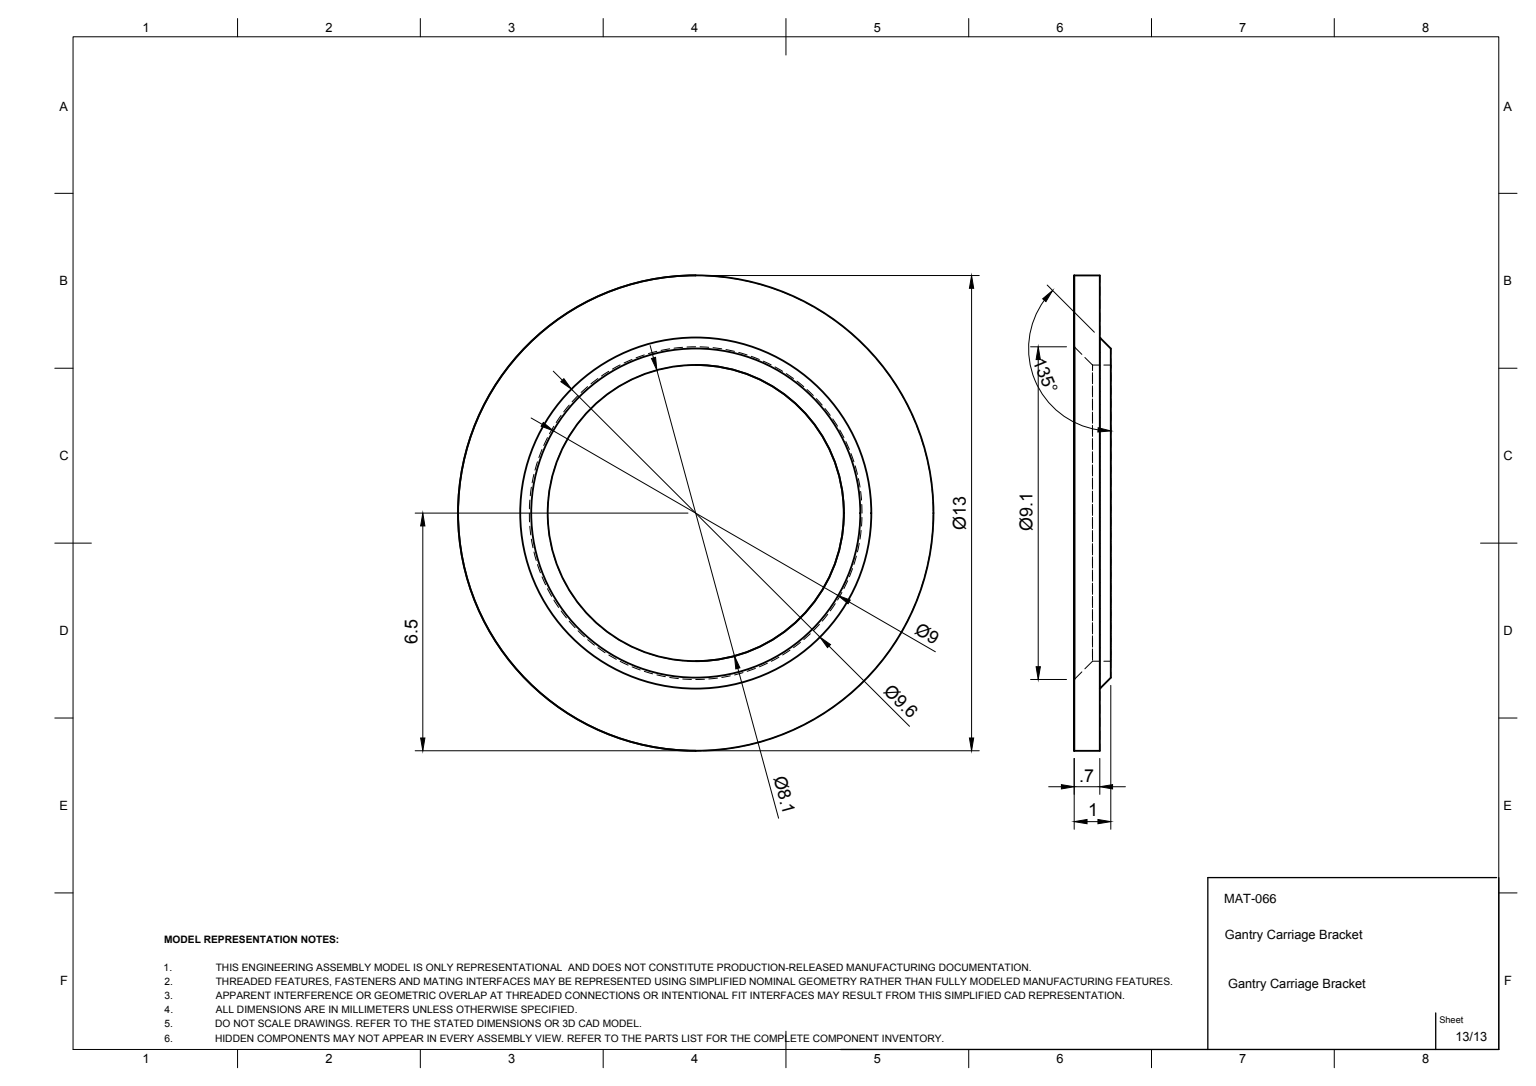
ISO-10303-21;
HEADER;
/* Generated by software containing ST-Developer
 * from STEP Tools, Inc. (www.steptools.com) 
 */

FILE_DESCRIPTION(
/* description */ ('CAx-IF Rec.Pracs.---Representation and Presentation of Product Manufa
cturing Information (PMI)---4.0---2014-10-13'),
/* implementation_level */ '2;1');

FILE_NAME(
/* name */ 'Gantry Carriage Bracket.step',
/* time_stamp */ '2026-10-24T15:58:00-07:00',
/* author */ (''),
/* organization */ (''),
/* preprocessor_version */ 'ST-DEVELOPER v20.2',
/* originating_system */ 'Autodesk Translation Framework v15.17.0.0',
/* authorisation */ '');

FILE_SCHEMA (('AP242_MANAGED_MODEL_BASED_3D_ENGINEERING_MIM_LF { 1 0 10303 442 2 1 4 }'));
ENDSEC;

DATA;
#10=MECHANICAL_DESIGN_GEOMETRIC_PRESENTATION_REPRESENTATION('',(#137),#8944);
#107=CONICAL_SURFACE('',#5788,0.0043,0.785398163397448);
#108=CONICAL_SURFACE('',#5794,0.0046499998960644,0.785398163397448);
#119=SHAPE_REPRESENTATION_RELATIONSHIP('SRR','None',#9002,#128);
#128=ADVANCED_BREP_SHAPE_REPRESENTATION('',(#146),#8943);
#137=STYLED_ITEM('',(#9052),#146);
#146=MANIFOLD_SOLID_BREP('Body1',#5158);
#236=CYLINDRICAL_SURFACE('',#5784,0.0065);
#237=CYLINDRICAL_SURFACE('',#5790,0.00405);
#305=FACE_BOUND('',#907,.T.);
#306=FACE_BOUND('',#910,.T.);
#307=FACE_BOUND('',#914,.T.);
#570=FACE_OUTER_BOUND('',#906,.T.);
#571=FACE_OUTER_BOUND('',#908,.T.);
#572=FACE_OUTER_BOUND('',#909,.T.);
#573=FACE_OUTER_BOUND('',#911,.T.);
#574=FACE_OUTER_BOUND('',#912,.T.);
#575=FACE_OUTER_BOUND('',#913,.T.);
#576=FACE_OUTER_BOUND('',#915,.T.);
#906=EDGE_LOOP('',(#4687));
#907=EDGE_LOOP('',(#4688));
#908=EDGE_LOOP('',(#4689,#4690,#4691,#4692));
#909=EDGE_LOOP('',(#4693));
#910=EDGE_LOOP('',(#4694));
#911=EDGE_LOOP('',(#4695,#4696,#4697,#4698));
#912=EDGE_LOOP('',(#4699,#4700,#4701,#4702));
#913=EDGE_LOOP('',(#4703));
#914=EDGE_LOOP('',(#4704));
#915=EDGE_LOOP('',(#4705,#4706,#4707,#4708));
#1165=CIRCLE('',#5782,0.00650000000001);
#1166=CIRCLE('',#5783,0.00479999989272164);
#1167=CIRCLE('',#5785,0.00650000000001);
#1168=CIRCLE('',#5787,0.00455000000001);
#1169=CIRCLE('',#5789,0.00405000000001);
#1170=CIRCLE('',#5791,0.00405000000001);
#1171=CIRCLE('',#5793,0.00449999989942716);
#1623=LINE('',#8881,#2078);
#1624=LINE('',#8889,#2079);
#1625=LINE('',#8892,#2080);
#1626=LINE('',#8898,#2081);
#2078=VECTOR('',#7320,0.0065);
#2079=VECTOR('',#7331,0.0043);
#2080=VECTOR('',#7334,0.00405);
#2081=VECTOR('',#7343,0.0046499998960644);
#2551=VERTEX_POINT('',#8875);
#2552=VERTEX_POINT('',#8877);
#2553=VERTEX_POINT('',#8880);
#2554=VERTEX_POINT('',#8884);
#2555=VERTEX_POINT('',#8887);
#2556=VERTEX_POINT('',#8891);
#2557=VERTEX_POINT('',#8895);
#3264=EDGE_CURVE('',#2551,#2551,#1165,.T.);
#3265=EDGE_CURVE('',#2552,#2552,#1166,.T.);
#3266=EDGE_CURVE('',#2551,#2553,#1623,.T.);
#3267=EDGE_CURVE('',#2553,#2553,#1167,.T.);
#3268=EDGE_CURVE('',#2554,#2554,#1168,.T.);
#3269=EDGE_CURVE('',#2555,#2555,#1169,.T.);
#3270=EDGE_CURVE('',#2555,#2554,#1624,.T.);
#3271=EDGE_CURVE('',#2555,#2556,#1625,.T.);
#3272=EDGE_CURVE('',#2556,#2556,#1170,.T.);
#3273=EDGE_CURVE('',#2557,#2557,#1171,.T.);
#3274=EDGE_CURVE('',#2552,#2557,#1626,.T.);
#4687=ORIENTED_EDGE('',*,*,#3264,.T.);
#4688=ORIENTED_EDGE('',*,*,#3265,.F.);
#4689=ORIENTED_EDGE('',*,*,#3264,.F.);
#4690=ORIENTED_EDGE('',*,*,#3266,.T.);
#4691=ORIENTED_EDGE('',*,*,#3267,.T.);
#4692=ORIENTED_EDGE('',*,*,#3266,.F.);
#4693=ORIENTED_EDGE('',*,*,#3267,.F.);
#4694=ORIENTED_EDGE('',*,*,#3268,.T.);
#4695=ORIENTED_EDGE('',*,*,#3269,.T.);
#4696=ORIENTED_EDGE('',*,*,#3270,.T.);
#4697=ORIENTED_EDGE('',*,*,#3268,.F.);
#4698=ORIENTED_EDGE('',*,*,#3270,.F.);
#4699=ORIENTED_EDGE('',*,*,#3269,.F.);
#4700=ORIENTED_EDGE('',*,*,#3271,.T.);
#4701=ORIENTED_EDGE('',*,*,#3272,.T.);
#4702=ORIENTED_EDGE('',*,*,#3271,.F.);
#4703=ORIENTED_EDGE('',*,*,#3273,.T.);
#4704=ORIENTED_EDGE('',*,*,#3272,.F.);
#4705=ORIENTED_EDGE('',*,*,#3265,.T.);
#4706=ORIENTED_EDGE('',*,*,#3274,.T.);
#4707=ORIENTED_EDGE('',*,*,#3273,.F.);
#4708=ORIENTED_EDGE('',*,*,#3274,.F.);
#4878=PLANE('',#5781);
#4879=PLANE('',#5786);
#4880=PLANE('',#5792);
#5143=ADVANCED_FACE('',(#570,#305),#4878,.F.);
#5144=ADVANCED_FACE('',(#571),#236,.T.);
#5145=ADVANCED_FACE('',(#572,#306),#4879,.F.);
#5146=ADVANCED_FACE('',(#573),#107,.F.);
#5147=ADVANCED_FACE('',(#574),#237,.F.);
#5148=ADVANCED_FACE('',(#575,#307),#4880,.F.);
#5149=ADVANCED_FACE('',(#576),#108,.T.);
#5158=CLOSED_SHELL('',(#5143,#5144,#5145,#5146,#5147,#5148,#5149));
#5780=AXIS2_PLACEMENT_3D('',#8873,#7310,#7311);
#5781=AXIS2_PLACEMENT_3D('',#8874,#7312,#7313);
#5782=AXIS2_PLACEMENT_3D('',#8876,#7314,#7315);
#5783=AXIS2_PLACEMENT_3D('',#8878,#7316,#7317);
#5784=AXIS2_PLACEMENT_3D('',#8879,#7318,#7319);
#5785=AXIS2_PLACEMENT_3D('',#8882,#7321,#7322);
#5786=AXIS2_PLACEMENT_3D('',#8883,#7323,#7324);
#5787=AXIS2_PLACEMENT_3D('',#8885,#7325,#7326);
#5788=AXIS2_PLACEMENT_3D('',#8886,#7327,#7328);
#5789=AXIS2_PLACEMENT_3D('',#8888,#7329,#7330);
#5790=AXIS2_PLACEMENT_3D('',#8890,#7332,#7333);
#5791=AXIS2_PLACEMENT_3D('',#8893,#7335,#7336);
#5792=AXIS2_PLACEMENT_3D('',#8894,#7337,#7338);
#5793=AXIS2_PLACEMENT_3D('',#8896,#7339,#7340);
#5794=AXIS2_PLACEMENT_3D('',#8897,#7341,#7342);
#7310=DIRECTION('axis',(0.,0.,1.));
#7311=DIRECTION('refdir',(1.,0.,0.));
#7312=DIRECTION('center_axis',(0.,-1.,0.));
#7313=DIRECTION('ref_axis',(1.,0.,0.));
#7314=DIRECTION('center_axis',(0.,1.,0.));
#7315=DIRECTION('ref_axis',(1.,0.,0.));
#7316=DIRECTION('center_axis',(0.,1.,0.));
#7317=DIRECTION('ref_axis',(1.,0.,0.));
#7318=DIRECTION('center_axis',(0.,1.,0.));
#7319=DIRECTION('ref_axis',(0.,0.,1.));
#7320=DIRECTION('',(0.,-1.,0.));
#7321=DIRECTION('center_axis',(0.,1.,0.));
#7322=DIRECTION('ref_axis',(1.,0.,0.));
#7323=DIRECTION('center_axis',(0.,1.,0.));
#7324=DIRECTION('ref_axis',(0.,0.,1.));
#7325=DIRECTION('center_axis',(0.,1.,0.));
#7326=DIRECTION('ref_axis',(1.,0.,0.));
#7327=DIRECTION('center_axis',(0.,-1.,0.));
#7328=DIRECTION('ref_axis',(0.,0.,1.));
#7329=DIRECTION('center_axis',(0.,1.,0.));
#7330=DIRECTION('ref_axis',(1.,0.,0.));
#7331=DIRECTION('',(8.65956056235493E-17,-0.707106781186548,-0.707106781186547));
#7332=DIRECTION('center_axis',(0.,1.,0.));
#7333=DIRECTION('ref_axis',(0.,0.,1.));
#7334=DIRECTION('',(0.,1.,0.));
#7335=DIRECTION('center_axis',(0.,1.,0.));
#7336=DIRECTION('ref_axis',(1.,0.,0.));
#7337=DIRECTION('center_axis',(0.,-1.,0.));
#7338=DIRECTION('ref_axis',(1.,0.,0.));
#7339=DIRECTION('center_axis',(0.,1.,0.));
#7340=DIRECTION('ref_axis',(1.,0.,0.));
#7341=DIRECTION('center_axis',(0.,-1.,0.));
#7342=DIRECTION('ref_axis',(0.,0.,1.));
#7343=DIRECTION('',(-8.65956056235493E-17,0.707106781186548,0.707106781186547));
#8873=CARTESIAN_POINT('',(0.,0.,0.));
#8874=CARTESIAN_POINT('Origin',(0.,0.0116999997384846,0.0065));
#8875=CARTESIAN_POINT('',(-7.9602041944578E-19,0.0116999997384946,-0.0065));
#8876=CARTESIAN_POINT('Origin',(0.,0.0116999997384946,0.));
#8877=CARTESIAN_POINT('',(5.87830450451699E-19,0.0116999997384846,-0.00479999989271167));
#8878=CARTESIAN_POINT('Origin',(0.,0.0116999997384946,0.));
#8879=CARTESIAN_POINT('Origin',(0.,0.0113499997351319,0.));
#8880=CARTESIAN_POINT('',(-7.9602041944578E-19,0.0109999997317891,-0.0065));
#8881=CARTESIAN_POINT('',(-7.9602041944578E-19,0.0113499997351319,-0.0065));
#8882=CARTESIAN_POINT('Origin',(0.,0.0109999997317891,0.));
#8883=CARTESIAN_POINT('Origin',(0.,0.0109999997317791,0.00455));
#8884=CARTESIAN_POINT('',(5.57214293612046E-19,0.0109999997317791,-0.00455));
#8885=CARTESIAN_POINT('Origin',(0.,0.0109999997317891,0.));
#8886=CARTESIAN_POINT('Origin',(0.,0.0112499997317791,0.));
#8887=CARTESIAN_POINT('',(4.95981953654678E-19,0.0114999997317791,-0.00405));
#8888=CARTESIAN_POINT('Origin',(0.,0.0114999997317891,0.));
#8889=CARTESIAN_POINT('',(5.26598123633362E-19,0.0112499997317791,-0.0043));
#8890=CARTESIAN_POINT('Origin',(0.,0.0117499997317791,0.));
#8891=CARTESIAN_POINT('',(-4.95981953654678E-19,0.0119999997317891,-0.00405));
#8892=CARTESIAN_POINT('',(-4.95981953654678E-19,0.0117499997317791,-0.00405));
#8893=CARTESIAN_POINT('Origin',(0.,0.0119999997317891,0.));
#8894=CARTESIAN_POINT('Origin',(0.,0.0119999997317791,0.00449999989941716));
#8895=CARTESIAN_POINT('',(5.51091047298466E-19,0.0119999997317791,-0.00449999989941718));
#8896=CARTESIAN_POINT('Origin',(0.,0.0119999997317891,0.));
#8897=CARTESIAN_POINT('Origin',(0.,0.0118499997351319,0.));
#8898=CARTESIAN_POINT('',(5.69460748875079E-19,0.0118499997351319,-0.0046499998960644));
#8931=UNCERTAINTY_MEASURE_WITH_UNIT(LENGTH_MEASURE(1.E-5),#8945,
'DISTANCE_ACCURACY_VALUE',
'Maximum model space distance between geometric entities at asserted c
onnectivities');
#8932=UNCERTAINTY_MEASURE_WITH_UNIT(LENGTH_MEASURE(1.E-5),#8945,
'DISTANCE_ACCURACY_VALUE',
'Maximum model space distance between geometric entities at asserted c
onnectivities');
#8943=(
GEOMETRIC_REPRESENTATION_CONTEXT(3)
GLOBAL_UNCERTAINTY_ASSIGNED_CONTEXT((#8931))
GLOBAL_UNIT_ASSIGNED_CONTEXT((#8945,#8946,#8947))
REPRESENTATION_CONTEXT('','3D')
);
#8944=(
GEOMETRIC_REPRESENTATION_CONTEXT(3)
GLOBAL_UNCERTAINTY_ASSIGNED_CONTEXT((#8932))
GLOBAL_UNIT_ASSIGNED_CONTEXT((#8945,#8946,#8947))
REPRESENTATION_CONTEXT('','3D')
);
#8945=(
LENGTH_UNIT()
NAMED_UNIT(*)
SI_UNIT($,.METRE.)
);
#8946=(
NAMED_UNIT(*)
PLANE_ANGLE_UNIT()
SI_UNIT($,.RADIAN.)
);
#8947=(
NAMED_UNIT(*)
SI_UNIT($,.STERADIAN.)
SOLID_ANGLE_UNIT()
);
#8958=SHAPE_DEFINITION_REPRESENTATION(#8969,#9002);
#8969=PRODUCT_DEFINITION_SHAPE('',$,#9014);
#9002=SHAPE_REPRESENTATION('',(#5780),#8943);
#9003=PRODUCT_DEFINITION_CONTEXT('part definition',#9038,'design');
#9014=PRODUCT_DEFINITION('Gantry Carriage Bracket',
'Gantry Carriage Bracket',#9025,#9003);
#9025=PRODUCT_DEFINITION_FORMATION('',$,#9050);
#9038=APPLICATION_CONTEXT('Managed model based 3d engineering');
#9039=PRODUCT_CONTEXT('part definition',#9038,'mechanical');
#9050=PRODUCT('Gantry Carriage Bracket','Gantry Carriage Bracket',
'LEGAL AND USAGE DISCLAIMER: this Data/Model is provided \X2\201C\X0\A
S IS\X2\201D\X0\ for informational and representational only. It is a 
geometric approximation and is NOT engineered, certified, or guarantee
d for dimensional accuracy, exact tolerances, or production-level prec
ision. Vendor disclaims all implied warranties including fitness for a
 particular purpose. DO NOT USE FOR DIRECT PHYSICAL MANUFACTURING, AUT
OMATED PRODUCTION, OR SAFETY-CRITICAL SYSTEMS without independent engi
neering verification and resolution of any design discrepancies.',(#9039));
#9052=PRESENTATION_STYLE_ASSIGNMENT((#9057));
#9057=SURFACE_STYLE_USAGE(.BOTH.,#9062);
#9062=SURFACE_SIDE_STYLE('',(#9067));
#9067=SURFACE_STYLE_FILL_AREA(#9072);
#9072=FILL_AREA_STYLE('Opaque(25,25,25)',(#9077));
#9077=FILL_AREA_STYLE_COLOUR('Opaque(25,25,25)',#9082);
#9082=COLOUR_RGB('Opaque(25,25,25)',0.0980392156862745,0.0980392156862745,
0.0980392156862745);
ENDSEC;
END-ISO-10303-21;
